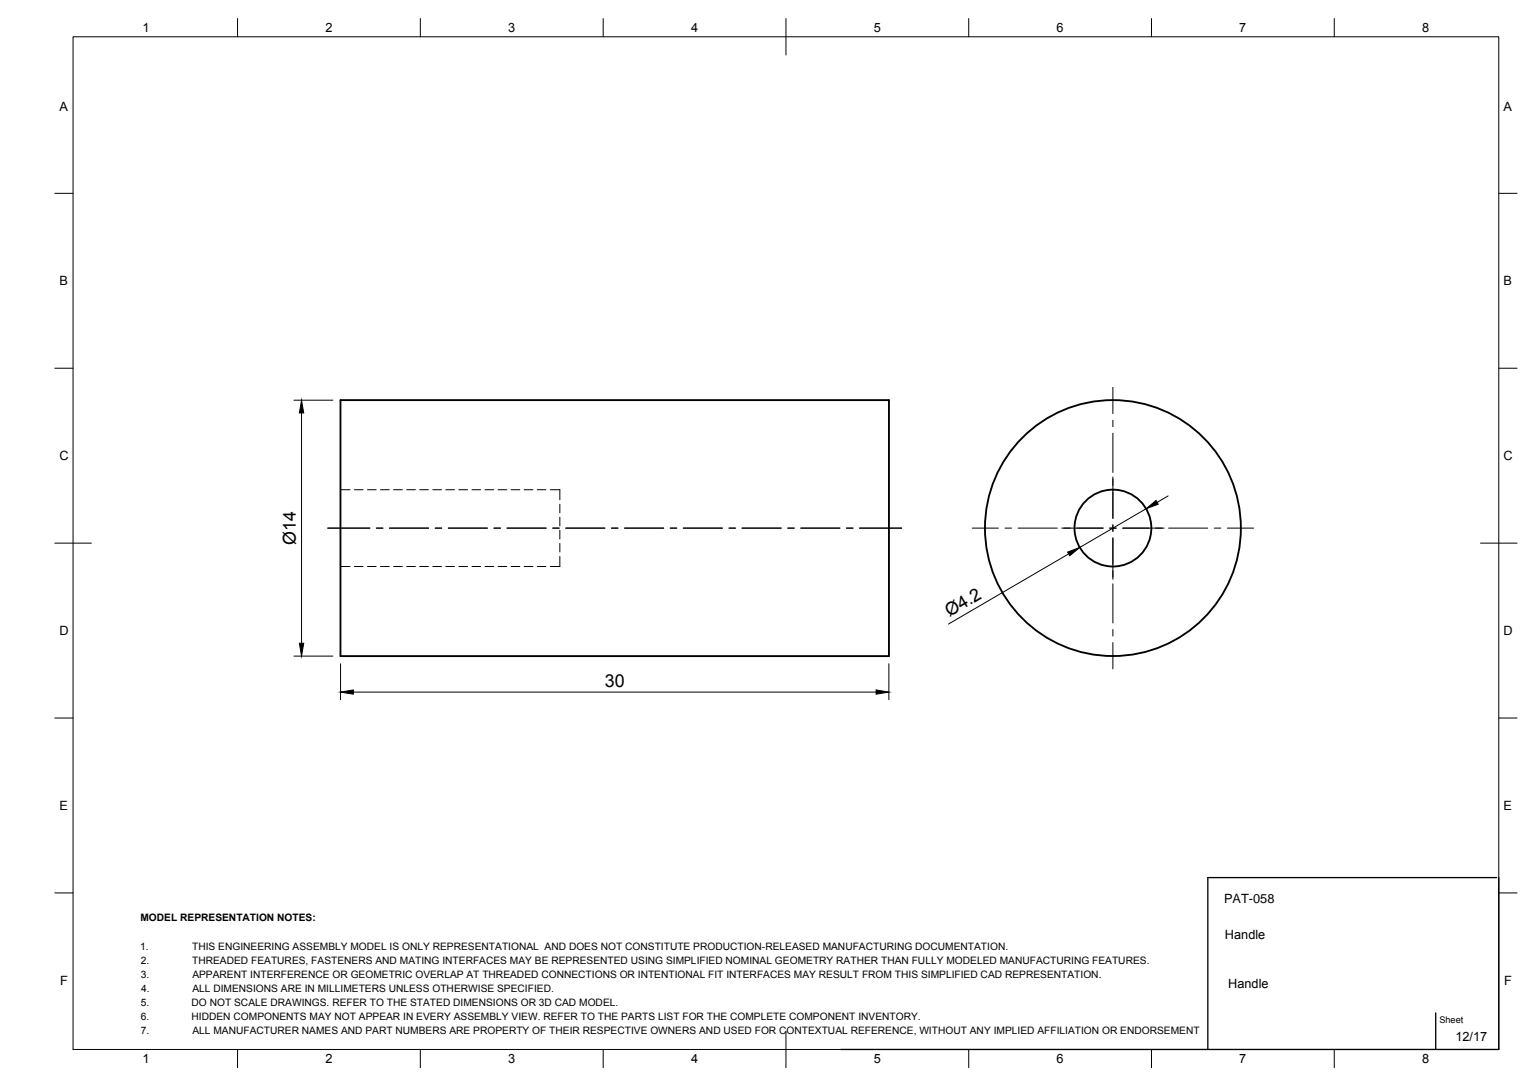
ISO-10303-21;
HEADER;
/* Generated by software containing ST-Developer
 * from STEP Tools, Inc. (www.steptools.com) 
 */

FILE_DESCRIPTION(
/* description */ ('Horizontal push-pull toggle clamp'),
/* implementation_level */ '2;1');

FILE_NAME(
/* name */ 'Handle.step',
/* time_stamp */ '2026-10-27T21:21:09-07:00',
/* author */ (''),
/* organization */ (''),
/* preprocessor_version */ 'ST-DEVELOPER v20.2',
/* originating_system */ 'Autodesk Translation Framework v15.17.0.0',
/* authorisation */ '');

FILE_SCHEMA (('AUTOMOTIVE_DESIGN { 1 0 10303 214 3 1 1 }'));
ENDSEC;

DATA;
#10=MECHANICAL_DESIGN_GEOMETRIC_PRESENTATION_REPRESENTATION('',(#187),#4791);
#161=SHAPE_REPRESENTATION_RELATIONSHIP('SRR','None',#4865,#174);
#174=ADVANCED_BREP_SHAPE_REPRESENTATION('',(#200),#4778);
#187=STYLED_ITEM('',(#5016),#200);
#200=MANIFOLD_SOLID_BREP('Body1',#2631);
#234=FACE_BOUND('',#600,.T.);
#303=PLANE('',#2885);
#304=PLANE('',#2889);
#305=PLANE('',#2890);
#421=FACE_OUTER_BOUND('',#596,.T.);
#422=FACE_OUTER_BOUND('',#597,.T.);
#423=FACE_OUTER_BOUND('',#598,.T.);
#424=FACE_OUTER_BOUND('',#599,.T.);
#425=FACE_OUTER_BOUND('',#601,.T.);
#596=EDGE_LOOP('',(#2077,#2078,#2079,#2080));
#597=EDGE_LOOP('',(#2081));
#598=EDGE_LOOP('',(#2082,#2083,#2084,#2085));
#599=EDGE_LOOP('',(#2086));
#600=EDGE_LOOP('',(#2087));
#601=EDGE_LOOP('',(#2088));
#740=CIRCLE('',#2883,0.21);
#741=CIRCLE('',#2884,0.21);
#742=CIRCLE('',#2887,0.7);
#743=CIRCLE('',#2888,0.7);
#913=LINE('',#4170,#1133);
#914=LINE('',#4177,#1134);
#1133=VECTOR('',#3381,0.21);
#1134=VECTOR('',#3390,0.7);
#1334=VERTEX_POINT('',#4167);
#1335=VERTEX_POINT('',#4169);
#1336=VERTEX_POINT('',#4174);
#1337=VERTEX_POINT('',#4176);
#1600=EDGE_CURVE('',#1334,#1334,#740,.T.);
#1601=EDGE_CURVE('',#1334,#1335,#913,.T.);
#1602=EDGE_CURVE('',#1335,#1335,#741,.T.);
#1603=EDGE_CURVE('',#1336,#1336,#742,.T.);
#1604=EDGE_CURVE('',#1336,#1337,#914,.T.);
#1605=EDGE_CURVE('',#1337,#1337,#743,.T.);
#2077=ORIENTED_EDGE('',*,*,#1600,.F.);
#2078=ORIENTED_EDGE('',*,*,#1601,.T.);
#2079=ORIENTED_EDGE('',*,*,#1602,.F.);
#2080=ORIENTED_EDGE('',*,*,#1601,.F.);
#2081=ORIENTED_EDGE('',*,*,#1600,.T.);
#2082=ORIENTED_EDGE('',*,*,#1603,.F.);
#2083=ORIENTED_EDGE('',*,*,#1604,.T.);
#2084=ORIENTED_EDGE('',*,*,#1605,.T.);
#2085=ORIENTED_EDGE('',*,*,#1604,.F.);
#2086=ORIENTED_EDGE('',*,*,#1603,.T.);
#2087=ORIENTED_EDGE('',*,*,#1602,.T.);
#2088=ORIENTED_EDGE('',*,*,#1605,.F.);
#2455=CYLINDRICAL_SURFACE('',#2882,0.21);
#2456=CYLINDRICAL_SURFACE('',#2886,0.7);
#2537=ADVANCED_FACE('',(#421),#2455,.F.);
#2538=ADVANCED_FACE('',(#422),#303,.T.);
#2539=ADVANCED_FACE('',(#423),#2456,.T.);
#2540=ADVANCED_FACE('',(#424,#234),#304,.T.);
#2541=ADVANCED_FACE('',(#425),#305,.F.);
#2631=CLOSED_SHELL('',(#2537,#2538,#2539,#2540,#2541));
#2881=AXIS2_PLACEMENT_3D('',#4165,#3375,#3376);
#2882=AXIS2_PLACEMENT_3D('',#4166,#3377,#3378);
#2883=AXIS2_PLACEMENT_3D('',#4168,#3379,#3380);
#2884=AXIS2_PLACEMENT_3D('',#4171,#3382,#3383);
#2885=AXIS2_PLACEMENT_3D('',#4172,#3384,#3385);
#2886=AXIS2_PLACEMENT_3D('',#4173,#3386,#3387);
#2887=AXIS2_PLACEMENT_3D('',#4175,#3388,#3389);
#2888=AXIS2_PLACEMENT_3D('',#4178,#3391,#3392);
#2889=AXIS2_PLACEMENT_3D('',#4179,#3393,#3394);
#2890=AXIS2_PLACEMENT_3D('',#4180,#3395,#3396);
#3375=DIRECTION('axis',(0.,0.,1.));
#3376=DIRECTION('refdir',(1.,0.,0.));
#3377=DIRECTION('center_axis',(0.,1.,0.));
#3378=DIRECTION('ref_axis',(1.,0.,0.));
#3379=DIRECTION('center_axis',(0.,1.,0.));
#3380=DIRECTION('ref_axis',(1.,0.,0.));
#3381=DIRECTION('',(0.,1.,0.));
#3382=DIRECTION('center_axis',(0.,-1.,0.));
#3383=DIRECTION('ref_axis',(1.,0.,0.));
#3384=DIRECTION('center_axis',(0.,1.,0.));
#3385=DIRECTION('ref_axis',(1.,0.,0.));
#3386=DIRECTION('center_axis',(0.,1.,0.));
#3387=DIRECTION('ref_axis',(1.,0.,0.));
#3388=DIRECTION('center_axis',(0.,1.,0.));
#3389=DIRECTION('ref_axis',(1.,0.,0.));
#3390=DIRECTION('',(0.,-1.,0.));
#3391=DIRECTION('center_axis',(0.,1.,0.));
#3392=DIRECTION('ref_axis',(1.,0.,0.));
#3393=DIRECTION('center_axis',(0.,1.,0.));
#3394=DIRECTION('ref_axis',(1.,0.,0.));
#3395=DIRECTION('center_axis',(0.,1.,0.));
#3396=DIRECTION('ref_axis',(1.,0.,0.));
#4165=CARTESIAN_POINT('',(0.,0.,0.));
#4166=CARTESIAN_POINT('Origin',(0.,-7.7,10.03));
#4167=CARTESIAN_POINT('',(-0.21,-7.7,10.03));
#4168=CARTESIAN_POINT('Origin',(0.,-7.7,10.03));
#4169=CARTESIAN_POINT('',(-0.21,-6.5,10.03));
#4170=CARTESIAN_POINT('',(-0.21,-7.7,10.03));
#4171=CARTESIAN_POINT('Origin',(0.,-6.5,10.03));
#4172=CARTESIAN_POINT('Origin',(0.,-7.7,10.03));
#4173=CARTESIAN_POINT('Origin',(0.,-9.5,10.03));
#4174=CARTESIAN_POINT('',(-0.7,-6.5,10.03));
#4175=CARTESIAN_POINT('Origin',(0.,-6.5,10.03));
#4176=CARTESIAN_POINT('',(-0.7,-9.5,10.03));
#4177=CARTESIAN_POINT('',(-0.7,-9.5,10.03));
#4178=CARTESIAN_POINT('Origin',(0.,-9.5,10.03));
#4179=CARTESIAN_POINT('Origin',(0.,-6.5,10.03));
#4180=CARTESIAN_POINT('Origin',(0.,-9.5,10.03));
#4759=UNCERTAINTY_MEASURE_WITH_UNIT(LENGTH_MEASURE(0.001),#4792,
'DISTANCE_ACCURACY_VALUE',
'Maximum model space distance between geometric entities at asserted c
onnectivities');
#4772=UNCERTAINTY_MEASURE_WITH_UNIT(LENGTH_MEASURE(0.001),#4792,
'DISTANCE_ACCURACY_VALUE',
'Maximum model space distance between geometric entities at asserted c
onnectivities');
#4778=(
GEOMETRIC_REPRESENTATION_CONTEXT(3)
GLOBAL_UNCERTAINTY_ASSIGNED_CONTEXT((#4759))
GLOBAL_UNIT_ASSIGNED_CONTEXT((#4792,#4794,#4795))
REPRESENTATION_CONTEXT('','3D')
);
#4791=(
GEOMETRIC_REPRESENTATION_CONTEXT(3)
GLOBAL_UNCERTAINTY_ASSIGNED_CONTEXT((#4772))
GLOBAL_UNIT_ASSIGNED_CONTEXT((#4792,#4794,#4795))
REPRESENTATION_CONTEXT('','3D')
);
#4792=(
LENGTH_UNIT()
NAMED_UNIT(*)
SI_UNIT(.CENTI.,.METRE.)
);
#4794=(
NAMED_UNIT(*)
PLANE_ANGLE_UNIT()
SI_UNIT($,.RADIAN.)
);
#4795=(
NAMED_UNIT(*)
SI_UNIT($,.STERADIAN.)
SOLID_ANGLE_UNIT()
);
#4801=SHAPE_DEFINITION_REPRESENTATION(#4819,#4865);
#4819=PRODUCT_DEFINITION_SHAPE('',$,#4884);
#4865=SHAPE_REPRESENTATION('',(#2881),#4778);
#4878=PRODUCT_DEFINITION_CONTEXT('part definition',#4934,'design');
#4884=PRODUCT_DEFINITION('Handle','Handle',#4902,#4878);
#4902=PRODUCT_DEFINITION_FORMATION('',$,#4941);
#4934=APPLICATION_CONTEXT(
'Core Data for Automotive Mechanical Design Process');
#4935=PRODUCT_CONTEXT('part definition',#4934,'mechanical');
#4941=PRODUCT('Handle','Handle','Handle',(#4935));
#5010=COLOUR_RGB('Sky Blue',0.24,0.69,0.87);
#5011=FILL_AREA_STYLE_COLOUR('',#5010);
#5012=FILL_AREA_STYLE('',(#5011));
#5013=SURFACE_STYLE_FILL_AREA(#5012);
#5014=SURFACE_SIDE_STYLE('',(#5013));
#5015=SURFACE_STYLE_USAGE(.BOTH.,#5014);
#5016=PRESENTATION_STYLE_ASSIGNMENT((#5015));
ENDSEC;
END-ISO-10303-21;
